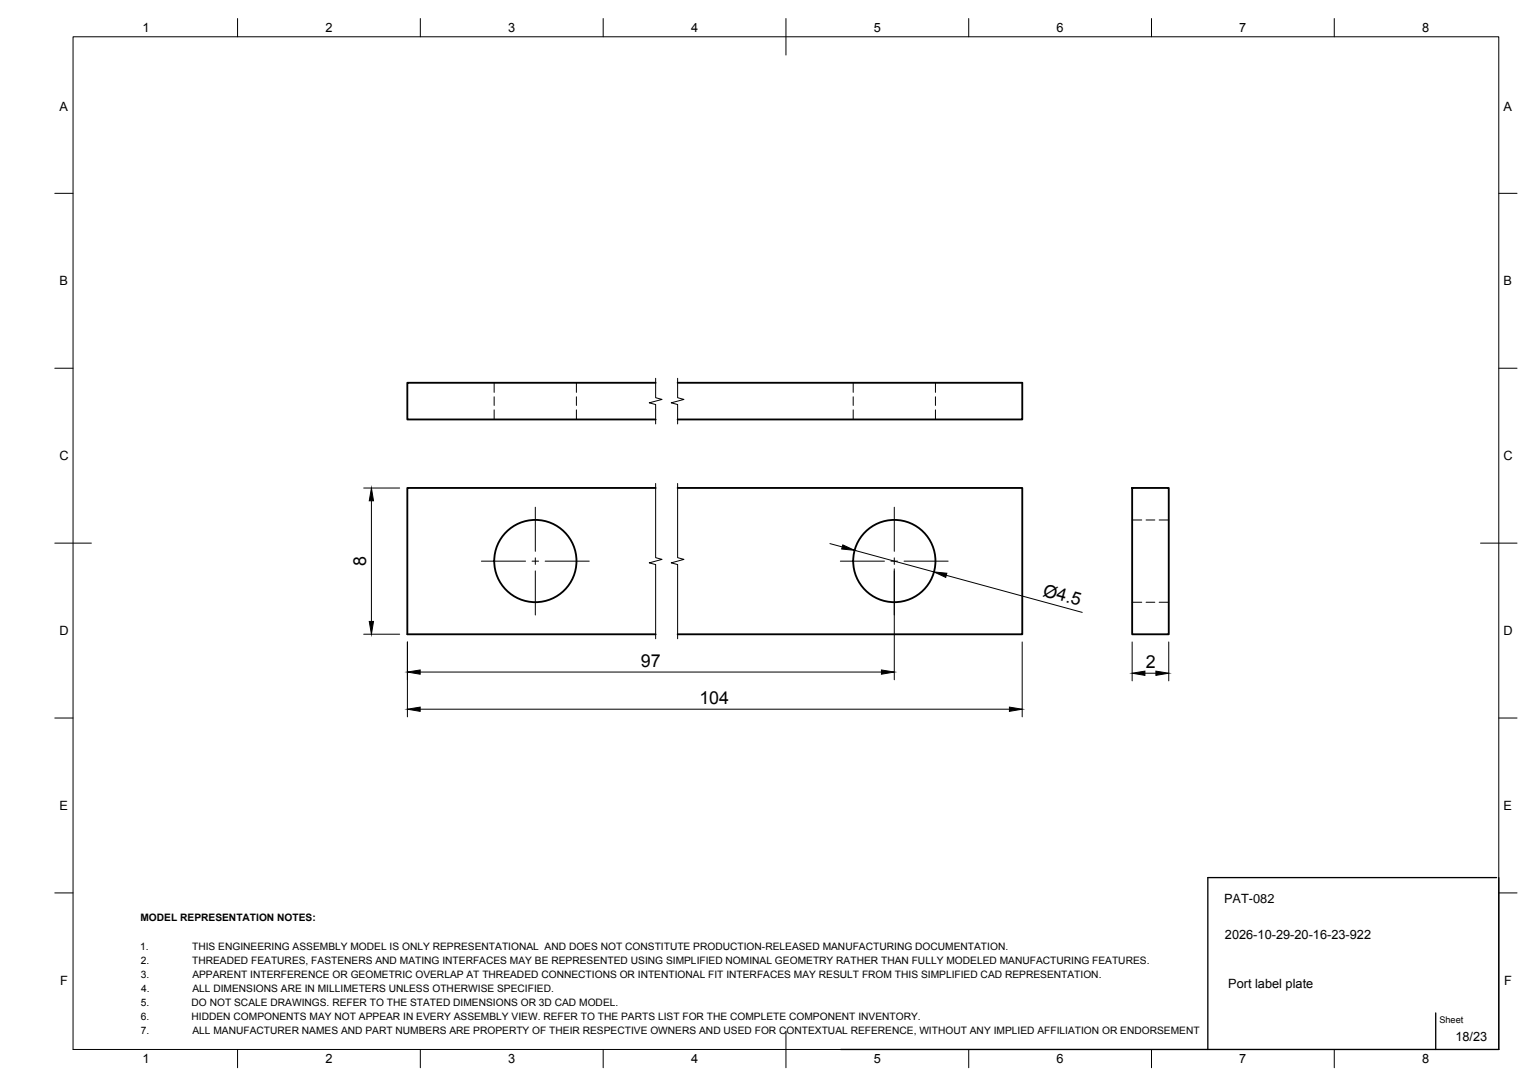
ISO-10303-21;
HEADER;
/* Generated by software containing ST-Developer
 * from STEP Tools, Inc. (www.steptools.com) 
 */

FILE_DESCRIPTION(
/* description */ ('PAT-082'),
/* implementation_level */ '2;1');

FILE_NAME(
/* name */ 'Port label plate.step',
/* time_stamp */ '2026-10-29T20:16:13-07:00',
/* author */ (''),
/* organization */ (''),
/* preprocessor_version */ 'ST-DEVELOPER v20.2',
/* originating_system */ 'Autodesk Translation Framework v15.17.0.0',
/* authorisation */ '');

FILE_SCHEMA (('AUTOMOTIVE_DESIGN { 1 0 10303 214 3 1 1 }'));
ENDSEC;

DATA;
#10=MECHANICAL_DESIGN_GEOMETRIC_PRESENTATION_REPRESENTATION('',(#256),#8266);
#212=SHAPE_REPRESENTATION_RELATIONSHIP('SRR','None',#8374,#234);
#234=ADVANCED_BREP_SHAPE_REPRESENTATION('',(#278),#8258);
#256=STYLED_ITEM('',(#8523),#278);
#278=MANIFOLD_SOLID_BREP('Body1',#4596);
#385=FACE_BOUND('',#1123,.T.);
#386=FACE_BOUND('',#1124,.T.);
#387=FACE_BOUND('',#1127,.T.);
#388=FACE_BOUND('',#1128,.T.);
#508=PLANE('',#5197);
#509=PLANE('',#5198);
#510=PLANE('',#5199);
#511=PLANE('',#5200);
#512=PLANE('',#5201);
#513=PLANE('',#5202);
#747=FACE_OUTER_BOUND('',#1120,.T.);
#748=FACE_OUTER_BOUND('',#1121,.T.);
#749=FACE_OUTER_BOUND('',#1122,.T.);
#750=FACE_OUTER_BOUND('',#1125,.T.);
#751=FACE_OUTER_BOUND('',#1126,.T.);
#752=FACE_OUTER_BOUND('',#1129,.T.);
#753=FACE_OUTER_BOUND('',#1130,.T.);
#754=FACE_OUTER_BOUND('',#1131,.T.);
#1120=EDGE_LOOP('',(#3854,#3855,#3856,#3857));
#1121=EDGE_LOOP('',(#3858,#3859,#3860,#3861));
#1122=EDGE_LOOP('',(#3862,#3863,#3864,#3865));
#1123=EDGE_LOOP('',(#3866));
#1124=EDGE_LOOP('',(#3867));
#1125=EDGE_LOOP('',(#3868,#3869,#3870,#3871));
#1126=EDGE_LOOP('',(#3872,#3873,#3874,#3875));
#1127=EDGE_LOOP('',(#3876));
#1128=EDGE_LOOP('',(#3877));
#1129=EDGE_LOOP('',(#3878,#3879,#3880,#3881));
#1130=EDGE_LOOP('',(#3882,#3883,#3884,#3885));
#1131=EDGE_LOOP('',(#3886,#3887,#3888,#3889));
#1457=LINE('',#7779,#1812);
#1458=LINE('',#7785,#1813);
#1459=LINE('',#7790,#1814);
#1460=LINE('',#7792,#1815);
#1461=LINE('',#7794,#1816);
#1462=LINE('',#7795,#1817);
#1463=LINE('',#7798,#1818);
#1464=LINE('',#7800,#1819);
#1465=LINE('',#7801,#1820);
#1466=LINE('',#7804,#1821);
#1467=LINE('',#7806,#1822);
#1468=LINE('',#7807,#1823);
#1469=LINE('',#7809,#1824);
#1470=LINE('',#7810,#1825);
#1812=VECTOR('',#6292,0.225);
#1813=VECTOR('',#6299,0.225);
#1814=VECTOR('',#6304,1.);
#1815=VECTOR('',#6305,1.);
#1816=VECTOR('',#6306,1.);
#1817=VECTOR('',#6307,1.);
#1818=VECTOR('',#6310,1.);
#1819=VECTOR('',#6311,1.);
#1820=VECTOR('',#6312,1.);
#1821=VECTOR('',#6315,1.);
#1822=VECTOR('',#6316,1.);
#1823=VECTOR('',#6317,1.);
#1824=VECTOR('',#6320,1.);
#1825=VECTOR('',#6321,1.);
#2095=CIRCLE('',#5192,0.225);
#2096=CIRCLE('',#5193,0.225);
#2097=CIRCLE('',#5195,0.225);
#2098=CIRCLE('',#5196,0.225);
#2401=VERTEX_POINT('',#7776);
#2402=VERTEX_POINT('',#7778);
#2403=VERTEX_POINT('',#7782);
#2404=VERTEX_POINT('',#7784);
#2405=VERTEX_POINT('',#7788);
#2406=VERTEX_POINT('',#7789);
#2407=VERTEX_POINT('',#7791);
#2408=VERTEX_POINT('',#7793);
#2409=VERTEX_POINT('',#7797);
#2410=VERTEX_POINT('',#7799);
#2411=VERTEX_POINT('',#7803);
#2412=VERTEX_POINT('',#7805);
#2903=EDGE_CURVE('',#2401,#2401,#2095,.T.);
#2904=EDGE_CURVE('',#2401,#2402,#1457,.T.);
#2905=EDGE_CURVE('',#2402,#2402,#2096,.T.);
#2906=EDGE_CURVE('',#2403,#2403,#2097,.T.);
#2907=EDGE_CURVE('',#2403,#2404,#1458,.T.);
#2908=EDGE_CURVE('',#2404,#2404,#2098,.T.);
#2909=EDGE_CURVE('',#2405,#2406,#1459,.T.);
#2910=EDGE_CURVE('',#2406,#2407,#1460,.T.);
#2911=EDGE_CURVE('',#2408,#2407,#1461,.T.);
#2912=EDGE_CURVE('',#2405,#2408,#1462,.T.);
#2913=EDGE_CURVE('',#2409,#2405,#1463,.T.);
#2914=EDGE_CURVE('',#2410,#2408,#1464,.T.);
#2915=EDGE_CURVE('',#2409,#2410,#1465,.T.);
#2916=EDGE_CURVE('',#2411,#2409,#1466,.T.);
#2917=EDGE_CURVE('',#2412,#2410,#1467,.T.);
#2918=EDGE_CURVE('',#2411,#2412,#1468,.T.);
#2919=EDGE_CURVE('',#2406,#2411,#1469,.T.);
#2920=EDGE_CURVE('',#2407,#2412,#1470,.T.);
#3854=ORIENTED_EDGE('',*,*,#2903,.F.);
#3855=ORIENTED_EDGE('',*,*,#2904,.T.);
#3856=ORIENTED_EDGE('',*,*,#2905,.F.);
#3857=ORIENTED_EDGE('',*,*,#2904,.F.);
#3858=ORIENTED_EDGE('',*,*,#2906,.F.);
#3859=ORIENTED_EDGE('',*,*,#2907,.T.);
#3860=ORIENTED_EDGE('',*,*,#2908,.F.);
#3861=ORIENTED_EDGE('',*,*,#2907,.F.);
#3862=ORIENTED_EDGE('',*,*,#2909,.T.);
#3863=ORIENTED_EDGE('',*,*,#2910,.T.);
#3864=ORIENTED_EDGE('',*,*,#2911,.F.);
#3865=ORIENTED_EDGE('',*,*,#2912,.F.);
#3866=ORIENTED_EDGE('',*,*,#2905,.T.);
#3867=ORIENTED_EDGE('',*,*,#2908,.T.);
#3868=ORIENTED_EDGE('',*,*,#2913,.T.);
#3869=ORIENTED_EDGE('',*,*,#2912,.T.);
#3870=ORIENTED_EDGE('',*,*,#2914,.F.);
#3871=ORIENTED_EDGE('',*,*,#2915,.F.);
#3872=ORIENTED_EDGE('',*,*,#2916,.T.);
#3873=ORIENTED_EDGE('',*,*,#2915,.T.);
#3874=ORIENTED_EDGE('',*,*,#2917,.F.);
#3875=ORIENTED_EDGE('',*,*,#2918,.F.);
#3876=ORIENTED_EDGE('',*,*,#2903,.T.);
#3877=ORIENTED_EDGE('',*,*,#2906,.T.);
#3878=ORIENTED_EDGE('',*,*,#2919,.T.);
#3879=ORIENTED_EDGE('',*,*,#2918,.T.);
#3880=ORIENTED_EDGE('',*,*,#2920,.F.);
#3881=ORIENTED_EDGE('',*,*,#2910,.F.);
#3882=ORIENTED_EDGE('',*,*,#2920,.T.);
#3883=ORIENTED_EDGE('',*,*,#2917,.T.);
#3884=ORIENTED_EDGE('',*,*,#2914,.T.);
#3885=ORIENTED_EDGE('',*,*,#2911,.T.);
#3886=ORIENTED_EDGE('',*,*,#2919,.F.);
#3887=ORIENTED_EDGE('',*,*,#2909,.F.);
#3888=ORIENTED_EDGE('',*,*,#2913,.F.);
#3889=ORIENTED_EDGE('',*,*,#2916,.F.);
#4292=CYLINDRICAL_SURFACE('',#5191,0.225);
#4293=CYLINDRICAL_SURFACE('',#5194,0.225);
#4486=ADVANCED_FACE('',(#747),#4292,.F.);
#4487=ADVANCED_FACE('',(#748),#4293,.F.);
#4488=ADVANCED_FACE('',(#749,#385,#386),#508,.T.);
#4489=ADVANCED_FACE('',(#750),#509,.T.);
#4490=ADVANCED_FACE('',(#751,#387,#388),#510,.T.);
#4491=ADVANCED_FACE('',(#752),#511,.T.);
#4492=ADVANCED_FACE('',(#753),#512,.T.);
#4493=ADVANCED_FACE('',(#754),#513,.F.);
#4596=CLOSED_SHELL('',(#4486,#4487,#4488,#4489,#4490,#4491,#4492,#4493));
#5190=AXIS2_PLACEMENT_3D('',#7774,#6286,#6287);
#5191=AXIS2_PLACEMENT_3D('',#7775,#6288,#6289);
#5192=AXIS2_PLACEMENT_3D('',#7777,#6290,#6291);
#5193=AXIS2_PLACEMENT_3D('',#7780,#6293,#6294);
#5194=AXIS2_PLACEMENT_3D('',#7781,#6295,#6296);
#5195=AXIS2_PLACEMENT_3D('',#7783,#6297,#6298);
#5196=AXIS2_PLACEMENT_3D('',#7786,#6300,#6301);
#5197=AXIS2_PLACEMENT_3D('',#7787,#6302,#6303);
#5198=AXIS2_PLACEMENT_3D('',#7796,#6308,#6309);
#5199=AXIS2_PLACEMENT_3D('',#7802,#6313,#6314);
#5200=AXIS2_PLACEMENT_3D('',#7808,#6318,#6319);
#5201=AXIS2_PLACEMENT_3D('',#7811,#6322,#6323);
#5202=AXIS2_PLACEMENT_3D('',#7812,#6324,#6325);
#6286=DIRECTION('axis',(0.,0.,1.));
#6287=DIRECTION('refdir',(1.,0.,0.));
#6288=DIRECTION('center_axis',(0.,1.,0.));
#6289=DIRECTION('ref_axis',(1.,0.,0.));
#6290=DIRECTION('center_axis',(0.,1.,0.));
#6291=DIRECTION('ref_axis',(1.,0.,0.));
#6292=DIRECTION('',(0.,1.,0.));
#6293=DIRECTION('center_axis',(0.,-1.,0.));
#6294=DIRECTION('ref_axis',(1.,0.,0.));
#6295=DIRECTION('center_axis',(0.,1.,0.));
#6296=DIRECTION('ref_axis',(1.,0.,0.));
#6297=DIRECTION('center_axis',(0.,1.,0.));
#6298=DIRECTION('ref_axis',(1.,0.,0.));
#6299=DIRECTION('',(0.,1.,0.));
#6300=DIRECTION('center_axis',(0.,-1.,0.));
#6301=DIRECTION('ref_axis',(1.,0.,0.));
#6302=DIRECTION('center_axis',(0.,1.,0.));
#6303=DIRECTION('ref_axis',(-1.,0.,0.));
#6304=DIRECTION('',(-1.,0.,0.));
#6305=DIRECTION('',(0.,0.,1.));
#6306=DIRECTION('',(-1.,0.,0.));
#6307=DIRECTION('',(0.,0.,1.));
#6308=DIRECTION('center_axis',(1.,0.,0.));
#6309=DIRECTION('ref_axis',(0.,1.,0.));
#6310=DIRECTION('',(0.,1.,0.));
#6311=DIRECTION('',(0.,1.,0.));
#6312=DIRECTION('',(0.,0.,1.));
#6313=DIRECTION('center_axis',(0.,-1.,0.));
#6314=DIRECTION('ref_axis',(1.,0.,0.));
#6315=DIRECTION('',(1.,0.,0.));
#6316=DIRECTION('',(1.,0.,0.));
#6317=DIRECTION('',(0.,0.,1.));
#6318=DIRECTION('center_axis',(-1.,0.,0.));
#6319=DIRECTION('ref_axis',(0.,-1.,0.));
#6320=DIRECTION('',(0.,-1.,0.));
#6321=DIRECTION('',(0.,-1.,0.));
#6322=DIRECTION('center_axis',(0.,0.,1.));
#6323=DIRECTION('ref_axis',(1.,0.,0.));
#6324=DIRECTION('center_axis',(0.,0.,1.));
#6325=DIRECTION('ref_axis',(1.,0.,0.));
#7774=CARTESIAN_POINT('',(0.,0.,0.));
#7775=CARTESIAN_POINT('Origin',(-4.5,-2.,4.));
#7776=CARTESIAN_POINT('',(-4.725,-1.95,4.));
#7777=CARTESIAN_POINT('Origin',(-4.5,-1.95,4.));
#7778=CARTESIAN_POINT('',(-4.725,-1.75,4.));
#7779=CARTESIAN_POINT('',(-4.725,-2.,4.));
#7780=CARTESIAN_POINT('Origin',(-4.5,-1.75,4.));
#7781=CARTESIAN_POINT('Origin',(4.5,-2.,4.));
#7782=CARTESIAN_POINT('',(4.275,-1.95,4.));
#7783=CARTESIAN_POINT('Origin',(4.5,-1.95,4.));
#7784=CARTESIAN_POINT('',(4.275,-1.75,4.));
#7785=CARTESIAN_POINT('',(4.275,-2.,4.));
#7786=CARTESIAN_POINT('Origin',(4.5,-1.75,4.));
#7787=CARTESIAN_POINT('Origin',(5.2,-1.75,3.6));
#7788=CARTESIAN_POINT('',(5.2,-1.75,3.6));
#7789=CARTESIAN_POINT('',(-5.2,-1.75,3.6));
#7790=CARTESIAN_POINT('',(5.2,-1.75,3.6));
#7791=CARTESIAN_POINT('',(-5.2,-1.75,4.4));
#7792=CARTESIAN_POINT('',(-5.2,-1.75,3.6));
#7793=CARTESIAN_POINT('',(5.2,-1.75,4.4));
#7794=CARTESIAN_POINT('',(5.2,-1.75,4.4));
#7795=CARTESIAN_POINT('',(5.2,-1.75,3.6));
#7796=CARTESIAN_POINT('Origin',(5.2,-1.95,3.6));
#7797=CARTESIAN_POINT('',(5.2,-1.95,3.6));
#7798=CARTESIAN_POINT('',(5.2,-1.95,3.6));
#7799=CARTESIAN_POINT('',(5.2,-1.95,4.4));
#7800=CARTESIAN_POINT('',(5.2,-1.95,4.4));
#7801=CARTESIAN_POINT('',(5.2,-1.95,3.6));
#7802=CARTESIAN_POINT('Origin',(-5.2,-1.95,3.6));
#7803=CARTESIAN_POINT('',(-5.2,-1.95,3.6));
#7804=CARTESIAN_POINT('',(-5.2,-1.95,3.6));
#7805=CARTESIAN_POINT('',(-5.2,-1.95,4.4));
#7806=CARTESIAN_POINT('',(-5.2,-1.95,4.4));
#7807=CARTESIAN_POINT('',(-5.2,-1.95,3.6));
#7808=CARTESIAN_POINT('Origin',(-5.2,-1.75,3.6));
#7809=CARTESIAN_POINT('',(-5.2,-1.75,3.6));
#7810=CARTESIAN_POINT('',(-5.2,-1.75,4.4));
#7811=CARTESIAN_POINT('Origin',(0.,-1.85,4.4));
#7812=CARTESIAN_POINT('Origin',(0.,-1.85,3.6));
#8233=UNCERTAINTY_MEASURE_WITH_UNIT(LENGTH_MEASURE(0.001),#8267,
'DISTANCE_ACCURACY_VALUE',
'Maximum model space distance between geometric entities at asserted c
onnectivities');
#8241=UNCERTAINTY_MEASURE_WITH_UNIT(LENGTH_MEASURE(0.001),#8267,
'DISTANCE_ACCURACY_VALUE',
'Maximum model space distance between geometric entities at asserted c
onnectivities');
#8258=(
GEOMETRIC_REPRESENTATION_CONTEXT(3)
GLOBAL_UNCERTAINTY_ASSIGNED_CONTEXT((#8233))
GLOBAL_UNIT_ASSIGNED_CONTEXT((#8267,#8269,#8270))
REPRESENTATION_CONTEXT('','3D')
);
#8266=(
GEOMETRIC_REPRESENTATION_CONTEXT(3)
GLOBAL_UNCERTAINTY_ASSIGNED_CONTEXT((#8241))
GLOBAL_UNIT_ASSIGNED_CONTEXT((#8267,#8269,#8270))
REPRESENTATION_CONTEXT('','3D')
);
#8267=(
LENGTH_UNIT()
NAMED_UNIT(*)
SI_UNIT(.CENTI.,.METRE.)
);
#8269=(
NAMED_UNIT(*)
PLANE_ANGLE_UNIT()
SI_UNIT($,.RADIAN.)
);
#8270=(
NAMED_UNIT(*)
SI_UNIT($,.STERADIAN.)
SOLID_ANGLE_UNIT()
);
#8287=SHAPE_DEFINITION_REPRESENTATION(#8311,#8374);
#8311=PRODUCT_DEFINITION_SHAPE('',$,#8399);
#8374=SHAPE_REPRESENTATION('',(#5190),#8258);
#8382=PRODUCT_DEFINITION_CONTEXT('part definition',#8456,'design');
#8399=PRODUCT_DEFINITION('Port label plate','Port label plate',
#8423,#8382);
#8423=PRODUCT_DEFINITION_FORMATION('',$,#8474);
#8456=APPLICATION_CONTEXT(
'Core Data for Automotive Mechanical Design Process');
#8457=PRODUCT_CONTEXT('part definition',#8456,'mechanical');
#8474=PRODUCT('Port label plate','Port label plate',
'Port label plate',(#8457));
#8517=COLOUR_RGB('Light Blue',0.38,0.62,0.78);
#8518=FILL_AREA_STYLE_COLOUR('',#8517);
#8519=FILL_AREA_STYLE('',(#8518));
#8520=SURFACE_STYLE_FILL_AREA(#8519);
#8521=SURFACE_SIDE_STYLE('',(#8520));
#8522=SURFACE_STYLE_USAGE(.BOTH.,#8521);
#8523=PRESENTATION_STYLE_ASSIGNMENT((#8522));
ENDSEC;
END-ISO-10303-21;
